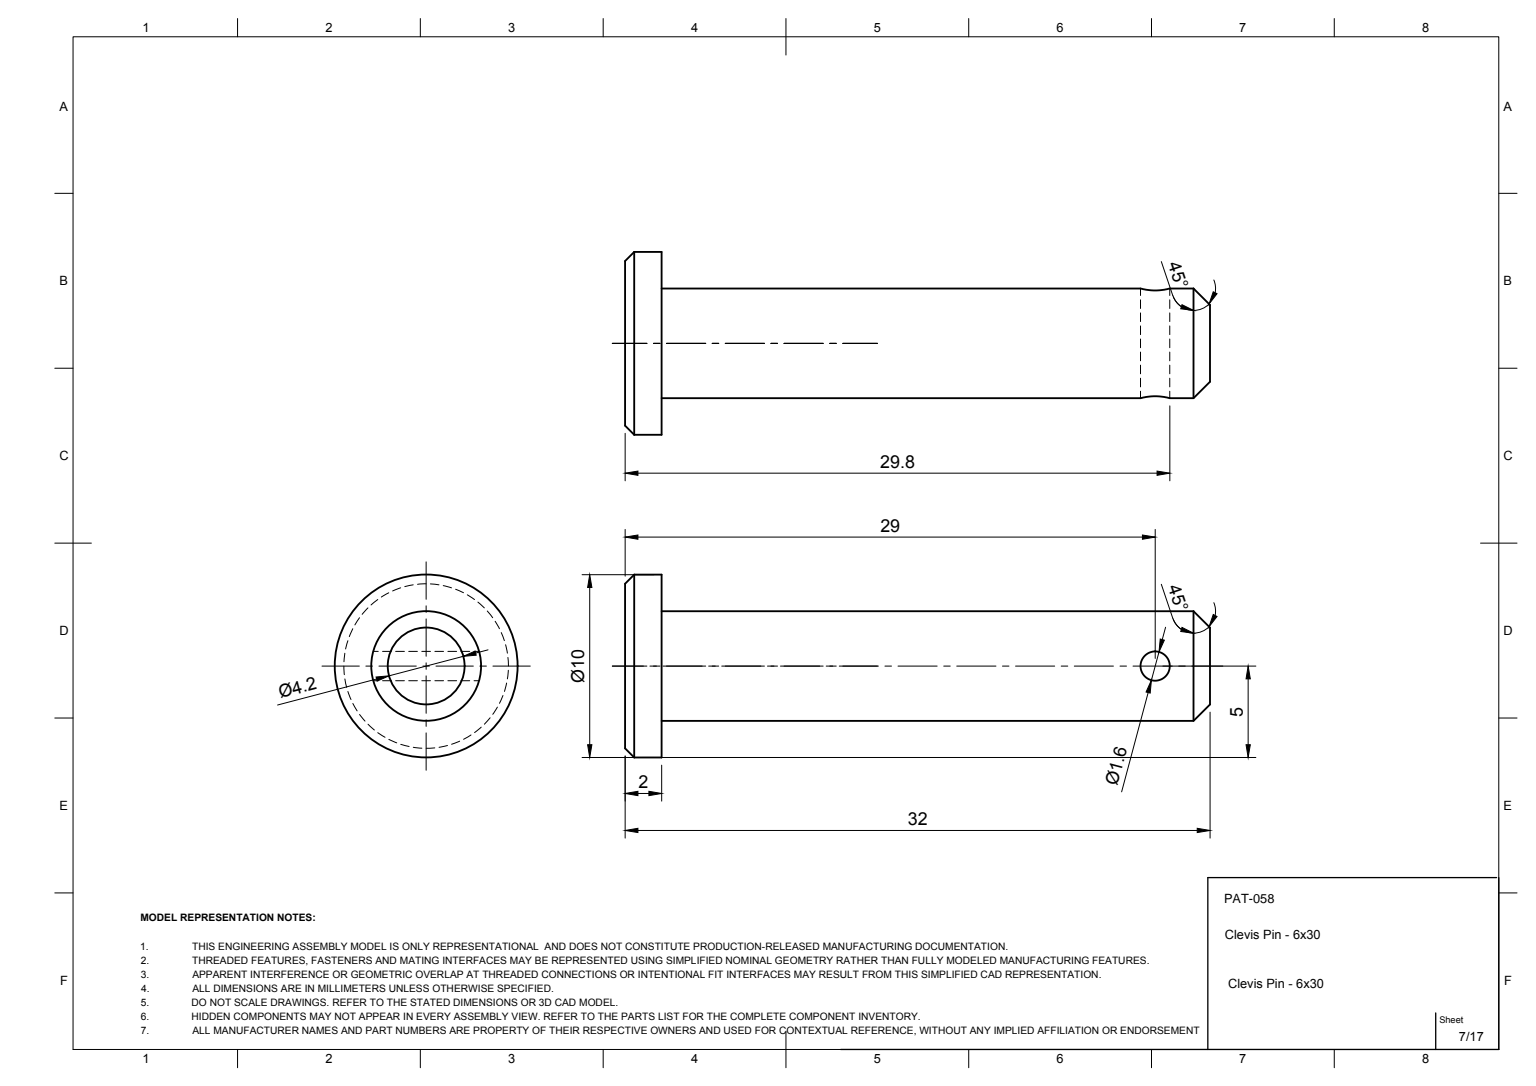
ISO-10303-21;
HEADER;
/* Generated by software containing ST-Developer
 * from STEP Tools, Inc. (www.steptools.com) 
 */

FILE_DESCRIPTION(
/* description */ ('Horizontal push-pull toggle clamp'),
/* implementation_level */ '2;1');

FILE_NAME(
/* name */ 'Clevis Pin - 6x30.step',
/* time_stamp */ '2026-10-27T21:21:09-07:00',
/* author */ (''),
/* organization */ (''),
/* preprocessor_version */ 'ST-DEVELOPER v20.2',
/* originating_system */ 'Autodesk Translation Framework v15.17.0.0',
/* authorisation */ '');

FILE_SCHEMA (('AUTOMOTIVE_DESIGN { 1 0 10303 214 3 1 1 }'));
ENDSEC;

DATA;
#10=MECHANICAL_DESIGN_GEOMETRIC_PRESENTATION_REPRESENTATION('',(#194),#4791);
#12=B_SPLINE_CURVE_WITH_KNOTS('',3,(#4522,#4523,#4524,#4525,#4526,#4527,
#4528,#4529,#4530,#4531),.UNSPECIFIED.,.F.,.F.,(4,2,2,2,4),(0.,0.0302963256060356,
0.0605926512120712,0.090883446720838,0.121174242229605),.UNSPECIFIED.);
#13=B_SPLINE_CURVE_WITH_KNOTS('',3,(#4534,#4535,#4536,#4537,#4538,#4539,
#4540,#4541,#4542,#4543,#4544,#4545,#4546,#4547,#4548,#4549,#4550,#4551,
#4552,#4553,#4554,#4555,#4556,#4557,#4558,#4559,#4560,#4561,#4562,#4563,
#4564,#4565,#4566,#4567),.UNSPECIFIED.,.T.,.F.,(4,2,2,2,2,2,2,2,2,2,2,2,
2,2,2,2,4),(0.,0.0302963256060358,0.0605926512120716,0.0908834467208383,
0.121174242229605,0.151465037738372,0.181755833247138,0.212052158853174,
0.24234848445921,0.272644810065246,0.302941135671282,0.333231931180048,
0.363522726688815,0.393813522197582,0.424104317706349,0.454400643312384,
0.48469696891842),.UNSPECIFIED.);
#14=B_SPLINE_CURVE_WITH_KNOTS('',3,(#4569,#4570,#4571,#4572,#4573,#4574,
#4575,#4576,#4577,#4578),.UNSPECIFIED.,.F.,.F.,(4,2,2,2,4),(0.363522726688815,
0.393813522197581,0.424104317706348,0.454400643312384,0.48469696891842),
 .UNSPECIFIED.);
#15=B_SPLINE_CURVE_WITH_KNOTS('',3,(#4579,#4580,#4581,#4582,#4583,#4584,
#4585,#4586,#4587,#4588,#4589,#4590,#4591,#4592,#4593,#4594,#4595,#4596),
 .UNSPECIFIED.,.F.,.F.,(4,2,2,2,2,2,2,2,4),(0.121174242229605,0.151465037738371,
0.181755833247138,0.212052158853174,0.24234848445921,0.272644810065246,
0.302941135671281,0.333231931180048,0.363522726688815),.UNSPECIFIED.);
#155=CONICAL_SURFACE('',#3003,0.475,0.785398163397448);
#156=CONICAL_SURFACE('',#3011,0.255,0.785398163397449);
#168=SHAPE_REPRESENTATION_RELATIONSHIP('SRR','None',#4874,#181);
#181=ADVANCED_BREP_SHAPE_REPRESENTATION('',(#206),#4787);
#194=STYLED_ITEM('',(#5023),#206);
#206=MANIFOLD_SOLID_BREP('Body1',#2639);
#249=FACE_BOUND('',#687,.T.);
#250=FACE_BOUND('',#689,.T.);
#352=PLANE('',#3001);
#353=PLANE('',#3007);
#354=PLANE('',#3013);
#492=FACE_OUTER_BOUND('',#682,.T.);
#493=FACE_OUTER_BOUND('',#683,.T.);
#494=FACE_OUTER_BOUND('',#684,.T.);
#495=FACE_OUTER_BOUND('',#685,.T.);
#496=FACE_OUTER_BOUND('',#686,.T.);
#497=FACE_OUTER_BOUND('',#688,.T.);
#498=FACE_OUTER_BOUND('',#690,.T.);
#499=FACE_OUTER_BOUND('',#691,.T.);
#682=EDGE_LOOP('',(#2363,#2364,#2365,#2366,#2367,#2368));
#683=EDGE_LOOP('',(#2369));
#684=EDGE_LOOP('',(#2370,#2371,#2372,#2373));
#685=EDGE_LOOP('',(#2374,#2375,#2376,#2377));
#686=EDGE_LOOP('',(#2378));
#687=EDGE_LOOP('',(#2379));
#688=EDGE_LOOP('',(#2380,#2381,#2382,#2383,#2384,#2385,#2386,#2387,#2388));
#689=EDGE_LOOP('',(#2389));
#690=EDGE_LOOP('',(#2390,#2391,#2392,#2393));
#691=EDGE_LOOP('',(#2394));
#777=CIRCLE('',#3002,0.45);
#778=CIRCLE('',#3004,0.5);
#779=CIRCLE('',#3006,0.5);
#780=CIRCLE('',#3008,0.3);
#781=CIRCLE('',#3010,0.3);
#782=CIRCLE('',#3012,0.21);
#1001=LINE('',#4533,#1221);
#1002=LINE('',#4603,#1222);
#1003=LINE('',#4607,#1223);
#1004=LINE('',#4614,#1224);
#1005=LINE('',#4615,#1225);
#1006=LINE('',#4619,#1226);
#1221=VECTOR('',#3703,0.08);
#1222=VECTOR('',#3712,0.475);
#1223=VECTOR('',#3717,0.5);
#1224=VECTOR('',#3726,0.3);
#1225=VECTOR('',#3727,0.3);
#1226=VECTOR('',#3732,0.255);
#1427=VERTEX_POINT('',#4520);
#1428=VERTEX_POINT('',#4521);
#1429=VERTEX_POINT('',#4532);
#1430=VERTEX_POINT('',#4568);
#1431=VERTEX_POINT('',#4598);
#1432=VERTEX_POINT('',#4601);
#1433=VERTEX_POINT('',#4605);
#1434=VERTEX_POINT('',#4609);
#1435=VERTEX_POINT('',#4612);
#1436=VERTEX_POINT('',#4617);
#1743=EDGE_CURVE('',#1427,#1428,#12,.T.);
#1744=EDGE_CURVE('',#1427,#1429,#1001,.T.);
#1745=EDGE_CURVE('',#1429,#1429,#13,.T.);
#1746=EDGE_CURVE('',#1430,#1427,#14,.T.);
#1747=EDGE_CURVE('',#1428,#1430,#15,.T.);
#1748=EDGE_CURVE('',#1431,#1431,#777,.T.);
#1749=EDGE_CURVE('',#1432,#1432,#778,.T.);
#1750=EDGE_CURVE('',#1432,#1431,#1002,.T.);
#1751=EDGE_CURVE('',#1433,#1433,#779,.T.);
#1752=EDGE_CURVE('',#1433,#1432,#1003,.T.);
#1753=EDGE_CURVE('',#1434,#1434,#780,.T.);
#1754=EDGE_CURVE('',#1435,#1435,#781,.T.);
#1755=EDGE_CURVE('',#1435,#1428,#1004,.T.);
#1756=EDGE_CURVE('',#1430,#1434,#1005,.T.);
#1757=EDGE_CURVE('',#1436,#1436,#782,.T.);
#1758=EDGE_CURVE('',#1436,#1435,#1006,.T.);
#2363=ORIENTED_EDGE('',*,*,#1743,.F.);
#2364=ORIENTED_EDGE('',*,*,#1744,.T.);
#2365=ORIENTED_EDGE('',*,*,#1745,.F.);
#2366=ORIENTED_EDGE('',*,*,#1744,.F.);
#2367=ORIENTED_EDGE('',*,*,#1746,.F.);
#2368=ORIENTED_EDGE('',*,*,#1747,.F.);
#2369=ORIENTED_EDGE('',*,*,#1748,.F.);
#2370=ORIENTED_EDGE('',*,*,#1749,.F.);
#2371=ORIENTED_EDGE('',*,*,#1750,.T.);
#2372=ORIENTED_EDGE('',*,*,#1748,.T.);
#2373=ORIENTED_EDGE('',*,*,#1750,.F.);
#2374=ORIENTED_EDGE('',*,*,#1751,.F.);
#2375=ORIENTED_EDGE('',*,*,#1752,.T.);
#2376=ORIENTED_EDGE('',*,*,#1749,.T.);
#2377=ORIENTED_EDGE('',*,*,#1752,.F.);
#2378=ORIENTED_EDGE('',*,*,#1751,.T.);
#2379=ORIENTED_EDGE('',*,*,#1753,.F.);
#2380=ORIENTED_EDGE('',*,*,#1754,.F.);
#2381=ORIENTED_EDGE('',*,*,#1755,.T.);
#2382=ORIENTED_EDGE('',*,*,#1747,.T.);
#2383=ORIENTED_EDGE('',*,*,#1756,.T.);
#2384=ORIENTED_EDGE('',*,*,#1753,.T.);
#2385=ORIENTED_EDGE('',*,*,#1756,.F.);
#2386=ORIENTED_EDGE('',*,*,#1746,.T.);
#2387=ORIENTED_EDGE('',*,*,#1743,.T.);
#2388=ORIENTED_EDGE('',*,*,#1755,.F.);
#2389=ORIENTED_EDGE('',*,*,#1745,.T.);
#2390=ORIENTED_EDGE('',*,*,#1757,.F.);
#2391=ORIENTED_EDGE('',*,*,#1758,.T.);
#2392=ORIENTED_EDGE('',*,*,#1754,.T.);
#2393=ORIENTED_EDGE('',*,*,#1758,.F.);
#2394=ORIENTED_EDGE('',*,*,#1757,.T.);
#2470=CYLINDRICAL_SURFACE('',#3000,0.08);
#2471=CYLINDRICAL_SURFACE('',#3005,0.5);
#2472=CYLINDRICAL_SURFACE('',#3009,0.3);
#2608=ADVANCED_FACE('',(#492),#2470,.F.);
#2609=ADVANCED_FACE('',(#493),#352,.T.);
#2610=ADVANCED_FACE('',(#494),#155,.T.);
#2611=ADVANCED_FACE('',(#495),#2471,.T.);
#2612=ADVANCED_FACE('',(#496,#249),#353,.T.);
#2613=ADVANCED_FACE('',(#497,#250),#2472,.T.);
#2614=ADVANCED_FACE('',(#498),#156,.T.);
#2615=ADVANCED_FACE('',(#499),#354,.T.);
#2639=CLOSED_SHELL('',(#2608,#2609,#2610,#2611,#2612,#2613,#2614,#2615));
#2999=AXIS2_PLACEMENT_3D('',#4518,#3699,#3700);
#3000=AXIS2_PLACEMENT_3D('',#4519,#3701,#3702);
#3001=AXIS2_PLACEMENT_3D('',#4597,#3704,#3705);
#3002=AXIS2_PLACEMENT_3D('',#4599,#3706,#3707);
#3003=AXIS2_PLACEMENT_3D('',#4600,#3708,#3709);
#3004=AXIS2_PLACEMENT_3D('',#4602,#3710,#3711);
#3005=AXIS2_PLACEMENT_3D('',#4604,#3713,#3714);
#3006=AXIS2_PLACEMENT_3D('',#4606,#3715,#3716);
#3007=AXIS2_PLACEMENT_3D('',#4608,#3718,#3719);
#3008=AXIS2_PLACEMENT_3D('',#4610,#3720,#3721);
#3009=AXIS2_PLACEMENT_3D('',#4611,#3722,#3723);
#3010=AXIS2_PLACEMENT_3D('',#4613,#3724,#3725);
#3011=AXIS2_PLACEMENT_3D('',#4616,#3728,#3729);
#3012=AXIS2_PLACEMENT_3D('',#4618,#3730,#3731);
#3013=AXIS2_PLACEMENT_3D('',#4620,#3733,#3734);
#3699=DIRECTION('axis',(0.,0.,1.));
#3700=DIRECTION('refdir',(1.,0.,0.));
#3701=DIRECTION('center_axis',(1.,0.,0.));
#3702=DIRECTION('ref_axis',(0.,0.,-1.));
#3703=DIRECTION('',(1.,0.,0.));
#3704=DIRECTION('center_axis',(0.,1.,0.));
#3705=DIRECTION('ref_axis',(0.,0.,1.));
#3706=DIRECTION('center_axis',(0.,-1.,0.));
#3707=DIRECTION('ref_axis',(1.,0.,0.));
#3708=DIRECTION('center_axis',(0.,-1.,0.));
#3709=DIRECTION('ref_axis',(1.,0.,0.));
#3710=DIRECTION('center_axis',(0.,-1.,0.));
#3711=DIRECTION('ref_axis',(1.,0.,0.));
#3712=DIRECTION('',(0.707106781186547,0.707106781186548,8.65956056235493E-17));
#3713=DIRECTION('center_axis',(0.,-1.,0.));
#3714=DIRECTION('ref_axis',(1.,0.,0.));
#3715=DIRECTION('center_axis',(0.,-1.,0.));
#3716=DIRECTION('ref_axis',(1.,0.,0.));
#3717=DIRECTION('',(0.,1.,0.));
#3718=DIRECTION('center_axis',(0.,-1.,0.));
#3719=DIRECTION('ref_axis',(0.,0.,-1.));
#3720=DIRECTION('center_axis',(0.,-1.,0.));
#3721=DIRECTION('ref_axis',(1.,0.,0.));
#3722=DIRECTION('center_axis',(0.,-1.,0.));
#3723=DIRECTION('ref_axis',(1.,0.,0.));
#3724=DIRECTION('center_axis',(0.,-1.,0.));
#3725=DIRECTION('ref_axis',(1.,0.,0.));
#3726=DIRECTION('',(0.,1.,0.));
#3727=DIRECTION('',(0.,1.,0.));
#3728=DIRECTION('center_axis',(0.,1.,0.));
#3729=DIRECTION('ref_axis',(1.,0.,0.));
#3730=DIRECTION('center_axis',(0.,-1.,0.));
#3731=DIRECTION('ref_axis',(1.,0.,0.));
#3732=DIRECTION('',(-0.707106781186548,0.707106781186547,-8.65956056235494E-17));
#3733=DIRECTION('center_axis',(0.,-1.,0.));
#3734=DIRECTION('ref_axis',(0.,0.,-1.));
#4518=CARTESIAN_POINT('',(0.,0.,0.));
#4519=CARTESIAN_POINT('Origin',(0.,-2.7,0.));
#4520=CARTESIAN_POINT('',(-0.289136645896019,-2.7,0.08));
#4521=CARTESIAN_POINT('',(-0.3,-2.78,-2.27065106771523E-17));
#4522=CARTESIAN_POINT('Ctrl Pts',(-0.289136645896019,-2.7,0.08));
#4523=CARTESIAN_POINT('Ctrl Pts',(-0.289136645896019,-2.71009877520201,
0.08));
#4524=CARTESIAN_POINT('Ctrl Pts',(-0.289720927595908,-2.72083518625944,
0.0779717130936404));
#4525=CARTESIAN_POINT('Ctrl Pts',(-0.291799203044223,-2.74052980652726,
0.0697927537456149));
#4526=CARTESIAN_POINT('Ctrl Pts',(-0.293259762986909,-2.74949254880105,
0.0636445361887959));
#4527=CARTESIAN_POINT('Ctrl Pts',(-0.295976783522942,-2.76364324458222,
0.0494938404076284));
#4528=CARTESIAN_POINT('Ctrl Pts',(-0.297414335384467,-2.76979246713824,
0.0405305642602551));
#4529=CARTESIAN_POINT('Ctrl Pts',(-0.299439403644655,-2.77797216257078,
0.0208340363410407));
#4530=CARTESIAN_POINT('Ctrl Pts',(-0.3,-2.78,0.0100969318362556));
#4531=CARTESIAN_POINT('Ctrl Pts',(-0.3,-2.78,5.20417042793042E-18));
#4532=CARTESIAN_POINT('',(0.289136645896019,-2.7,0.08));
#4533=CARTESIAN_POINT('',(0.,-2.7,0.08));
#4534=CARTESIAN_POINT('Ctrl Pts',(0.289136645896019,-2.7,0.08));
#4535=CARTESIAN_POINT('Ctrl Pts',(0.289136645896019,-2.68990122479799,0.08));
#4536=CARTESIAN_POINT('Ctrl Pts',(0.289720927595908,-2.67916481374056,0.0779717130936404));
#4537=CARTESIAN_POINT('Ctrl Pts',(0.291799203044223,-2.65947019347274,0.0697927537456147));
#4538=CARTESIAN_POINT('Ctrl Pts',(0.293259762986909,-2.65050745119895,0.0636445361887959));
#4539=CARTESIAN_POINT('Ctrl Pts',(0.295976783522942,-2.63635675541778,0.0494938404076283));
#4540=CARTESIAN_POINT('Ctrl Pts',(0.297414335384467,-2.63020753286176,0.0405305642602551));
#4541=CARTESIAN_POINT('Ctrl Pts',(0.299439403644655,-2.62202783742922,0.0208340363410406));
#4542=CARTESIAN_POINT('Ctrl Pts',(0.3,-2.62,0.0100969318362555));
#4543=CARTESIAN_POINT('Ctrl Pts',(0.3,-2.62,-0.0100969318362556));
#4544=CARTESIAN_POINT('Ctrl Pts',(0.299439403644655,-2.62202783742922,-0.0208340363410406));
#4545=CARTESIAN_POINT('Ctrl Pts',(0.297414335384467,-2.63020753286176,-0.0405305642602551));
#4546=CARTESIAN_POINT('Ctrl Pts',(0.295976783522942,-2.63635675541778,-0.0494938404076283));
#4547=CARTESIAN_POINT('Ctrl Pts',(0.293259762986909,-2.65050745119895,-0.0636445361887959));
#4548=CARTESIAN_POINT('Ctrl Pts',(0.291799203044223,-2.65947019347274,-0.0697927537456147));
#4549=CARTESIAN_POINT('Ctrl Pts',(0.289720927595908,-2.67916481374056,-0.0779717130936403));
#4550=CARTESIAN_POINT('Ctrl Pts',(0.289136645896019,-2.68990122479799,-0.08));
#4551=CARTESIAN_POINT('Ctrl Pts',(0.289136645896019,-2.71009877520201,-0.08));
#4552=CARTESIAN_POINT('Ctrl Pts',(0.289720927595908,-2.72083518625944,-0.0779717130936404));
#4553=CARTESIAN_POINT('Ctrl Pts',(0.291799203044223,-2.74052980652726,-0.0697927537456147));
#4554=CARTESIAN_POINT('Ctrl Pts',(0.293259762986909,-2.74949254880105,-0.0636445361887959));
#4555=CARTESIAN_POINT('Ctrl Pts',(0.295976783522942,-2.76364324458222,-0.0494938404076283));
#4556=CARTESIAN_POINT('Ctrl Pts',(0.297414335384467,-2.76979246713824,-0.0405305642602551));
#4557=CARTESIAN_POINT('Ctrl Pts',(0.299439403644655,-2.77797216257078,-0.0208340363410406));
#4558=CARTESIAN_POINT('Ctrl Pts',(0.3,-2.78,-0.0100969318362555));
#4559=CARTESIAN_POINT('Ctrl Pts',(0.3,-2.78,0.0100969318362556));
#4560=CARTESIAN_POINT('Ctrl Pts',(0.299439403644655,-2.77797216257078,0.0208340363410407));
#4561=CARTESIAN_POINT('Ctrl Pts',(0.297414335384467,-2.76979246713824,0.0405305642602551));
#4562=CARTESIAN_POINT('Ctrl Pts',(0.295976783522942,-2.76364324458222,0.0494938404076284));
#4563=CARTESIAN_POINT('Ctrl Pts',(0.293259762986909,-2.74949254880105,0.0636445361887959));
#4564=CARTESIAN_POINT('Ctrl Pts',(0.291799203044223,-2.74052980652726,0.0697927537456149));
#4565=CARTESIAN_POINT('Ctrl Pts',(0.289720927595908,-2.72083518625944,0.0779717130936404));
#4566=CARTESIAN_POINT('Ctrl Pts',(0.289136645896019,-2.71009877520201,0.08));
#4567=CARTESIAN_POINT('Ctrl Pts',(0.289136645896019,-2.7,0.08));
#4568=CARTESIAN_POINT('',(-0.3,-2.62,-3.65842984849668E-17));
#4569=CARTESIAN_POINT('Ctrl Pts',(-0.3,-2.62,-3.81639164714898E-17));
#4570=CARTESIAN_POINT('Ctrl Pts',(-0.3,-2.62,0.0100969318362555));
#4571=CARTESIAN_POINT('Ctrl Pts',(-0.299439403644655,-2.62202783742922,
0.0208340363410406));
#4572=CARTESIAN_POINT('Ctrl Pts',(-0.297414335384467,-2.63020753286176,
0.040530564260255));
#4573=CARTESIAN_POINT('Ctrl Pts',(-0.295976783522942,-2.63635675541778,
0.0494938404076283));
#4574=CARTESIAN_POINT('Ctrl Pts',(-0.293259762986909,-2.65050745119895,
0.0636445361887959));
#4575=CARTESIAN_POINT('Ctrl Pts',(-0.291799203044223,-2.65947019347274,
0.0697927537456147));
#4576=CARTESIAN_POINT('Ctrl Pts',(-0.289720927595908,-2.67916481374056,
0.0779717130936404));
#4577=CARTESIAN_POINT('Ctrl Pts',(-0.289136645896019,-2.68990122479799,
0.08));
#4578=CARTESIAN_POINT('Ctrl Pts',(-0.289136645896019,-2.7,0.08));
#4579=CARTESIAN_POINT('Ctrl Pts',(-0.3,-2.78,-6.93889390390723E-18));
#4580=CARTESIAN_POINT('Ctrl Pts',(-0.3,-2.78,-0.0100969318362556));
#4581=CARTESIAN_POINT('Ctrl Pts',(-0.299439403644655,-2.77797216257078,
-0.0208340363410406));
#4582=CARTESIAN_POINT('Ctrl Pts',(-0.297414335384467,-2.76979246713824,
-0.0405305642602551));
#4583=CARTESIAN_POINT('Ctrl Pts',(-0.295976783522942,-2.76364324458222,
-0.0494938404076283));
#4584=CARTESIAN_POINT('Ctrl Pts',(-0.293259762986909,-2.74949254880105,
-0.0636445361887959));
#4585=CARTESIAN_POINT('Ctrl Pts',(-0.291799203044223,-2.74052980652726,
-0.0697927537456147));
#4586=CARTESIAN_POINT('Ctrl Pts',(-0.289720927595908,-2.72083518625944,
-0.0779717130936403));
#4587=CARTESIAN_POINT('Ctrl Pts',(-0.289136645896019,-2.71009877520201,
-0.08));
#4588=CARTESIAN_POINT('Ctrl Pts',(-0.289136645896019,-2.68990122479799,
-0.08));
#4589=CARTESIAN_POINT('Ctrl Pts',(-0.289720927595908,-2.67916481374056,
-0.0779717130936403));
#4590=CARTESIAN_POINT('Ctrl Pts',(-0.291799203044223,-2.65947019347274,
-0.0697927537456147));
#4591=CARTESIAN_POINT('Ctrl Pts',(-0.293259762986909,-2.65050745119895,
-0.0636445361887959));
#4592=CARTESIAN_POINT('Ctrl Pts',(-0.295976783522942,-2.63635675541778,
-0.0494938404076283));
#4593=CARTESIAN_POINT('Ctrl Pts',(-0.297414335384467,-2.63020753286176,
-0.0405305642602551));
#4594=CARTESIAN_POINT('Ctrl Pts',(-0.299439403644655,-2.62202783742922,
-0.0208340363410406));
#4595=CARTESIAN_POINT('Ctrl Pts',(-0.3,-2.62,-0.0100969318362556));
#4596=CARTESIAN_POINT('Ctrl Pts',(-0.3,-2.62,-1.56125112837913E-17));
#4597=CARTESIAN_POINT('Origin',(0.45,0.2,0.));
#4598=CARTESIAN_POINT('',(-0.45,0.2,-5.51091059616309E-17));
#4599=CARTESIAN_POINT('Origin',(0.,0.2,0.));
#4600=CARTESIAN_POINT('Origin',(0.,0.175,0.));
#4601=CARTESIAN_POINT('',(-0.5,0.15,-6.12323399573676E-17));
#4602=CARTESIAN_POINT('Origin',(0.,0.15,0.));
#4603=CARTESIAN_POINT('',(-0.475,0.175,-5.81707229594993E-17));
#4604=CARTESIAN_POINT('Origin',(0.,0.0750000000000002,0.));
#4605=CARTESIAN_POINT('',(-0.5,0.,-6.12323399573677E-17));
#4606=CARTESIAN_POINT('Origin',(0.,0.,0.));
#4607=CARTESIAN_POINT('',(-0.5,0.0750000000000002,-6.12323399573677E-17));
#4608=CARTESIAN_POINT('Origin',(0.3,0.,0.));
#4609=CARTESIAN_POINT('',(-0.3,0.,-3.67394039744206E-17));
#4610=CARTESIAN_POINT('Origin',(0.,0.,0.));
#4611=CARTESIAN_POINT('Origin',(0.,-1.455,0.));
#4612=CARTESIAN_POINT('',(-0.3,-2.91,-3.67394039744206E-17));
#4613=CARTESIAN_POINT('Origin',(0.,-2.91,0.));
#4614=CARTESIAN_POINT('',(-0.3,-1.455,-3.67394039744206E-17));
#4615=CARTESIAN_POINT('',(-0.3,-1.455,-3.67394039744206E-17));
#4616=CARTESIAN_POINT('Origin',(0.,-2.955,0.));
#4617=CARTESIAN_POINT('',(-0.21,-3.,-2.57175827820944E-17));
#4618=CARTESIAN_POINT('Origin',(0.,-3.,0.));
#4619=CARTESIAN_POINT('',(-0.255,-2.955,-3.12284933782575E-17));
#4620=CARTESIAN_POINT('Origin',(0.,-3.,0.));
#4768=UNCERTAINTY_MEASURE_WITH_UNIT(LENGTH_MEASURE(0.001),#4792,
'DISTANCE_ACCURACY_VALUE',
'Maximum model space distance between geometric entities at asserted c
onnectivities');
#4772=UNCERTAINTY_MEASURE_WITH_UNIT(LENGTH_MEASURE(0.001),#4792,
'DISTANCE_ACCURACY_VALUE',
'Maximum model space distance between geometric entities at asserted c
onnectivities');
#4787=(
GEOMETRIC_REPRESENTATION_CONTEXT(3)
GLOBAL_UNCERTAINTY_ASSIGNED_CONTEXT((#4768))
GLOBAL_UNIT_ASSIGNED_CONTEXT((#4792,#4794,#4795))
REPRESENTATION_CONTEXT('','3D')
);
#4791=(
GEOMETRIC_REPRESENTATION_CONTEXT(3)
GLOBAL_UNCERTAINTY_ASSIGNED_CONTEXT((#4772))
GLOBAL_UNIT_ASSIGNED_CONTEXT((#4792,#4794,#4795))
REPRESENTATION_CONTEXT('','3D')
);
#4792=(
LENGTH_UNIT()
NAMED_UNIT(*)
SI_UNIT(.CENTI.,.METRE.)
);
#4794=(
NAMED_UNIT(*)
PLANE_ANGLE_UNIT()
SI_UNIT($,.RADIAN.)
);
#4795=(
NAMED_UNIT(*)
SI_UNIT($,.STERADIAN.)
SOLID_ANGLE_UNIT()
);
#4810=SHAPE_DEFINITION_REPRESENTATION(#4829,#4874);
#4829=PRODUCT_DEFINITION_SHAPE('',$,#4893);
#4874=SHAPE_REPRESENTATION('',(#2999),#4787);
#4878=PRODUCT_DEFINITION_CONTEXT('part definition',#4934,'design');
#4893=PRODUCT_DEFINITION('Clevis Pin - 6x30','Clevis Pin - 6x30',#4911,
#4878);
#4911=PRODUCT_DEFINITION_FORMATION('',$,#4950);
#4934=APPLICATION_CONTEXT(
'Core Data for Automotive Mechanical Design Process');
#4935=PRODUCT_CONTEXT('part definition',#4934,'mechanical');
#4950=PRODUCT('Clevis Pin - 6x30','Clevis Pin - 6x30',
'Clevis Pin - 6x30',(#4935));
#5017=COLOUR_RGB('Grey',0.48,0.52,0.57);
#5018=FILL_AREA_STYLE_COLOUR('',#5017);
#5019=FILL_AREA_STYLE('',(#5018));
#5020=SURFACE_STYLE_FILL_AREA(#5019);
#5021=SURFACE_SIDE_STYLE('',(#5020));
#5022=SURFACE_STYLE_USAGE(.BOTH.,#5021);
#5023=PRESENTATION_STYLE_ASSIGNMENT((#5022));
ENDSEC;
END-ISO-10303-21;
